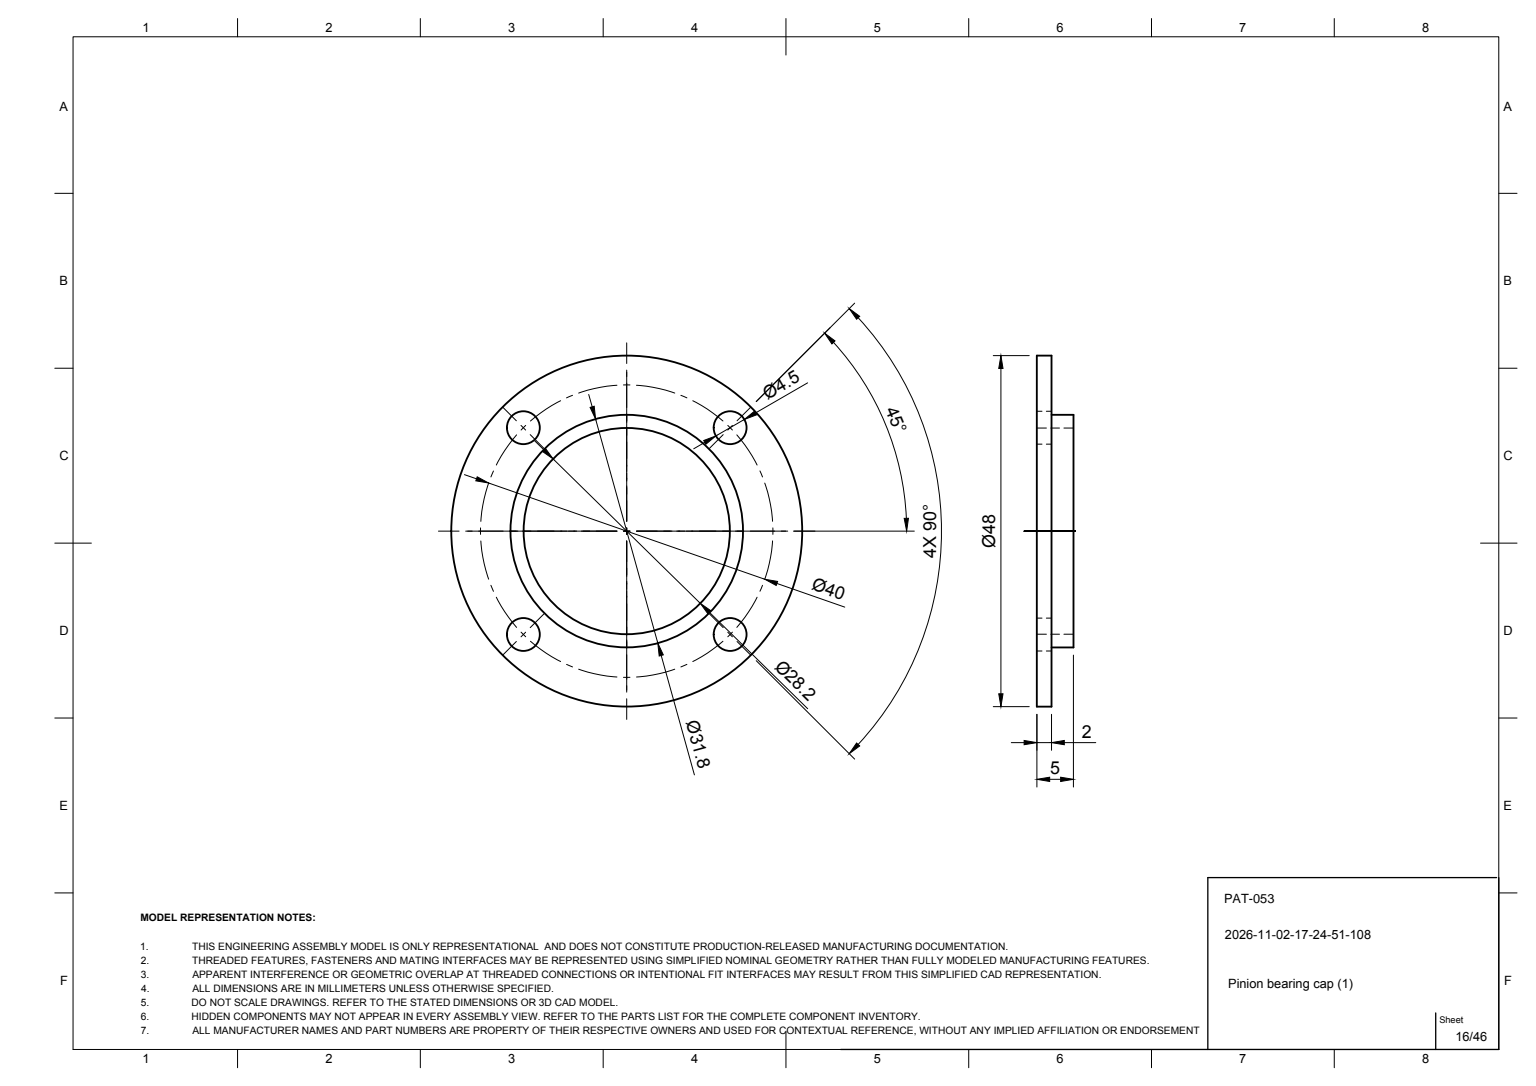
ISO-10303-21;
HEADER;
/* Generated by software containing ST-Developer
 * from STEP Tools, Inc. (www.steptools.com) 
 */

FILE_DESCRIPTION(
/* description */ ('Hand-operated arbor press'),
/* implementation_level */ '2;1');

FILE_NAME(
/* name */ 'Pinion bearing cap (1).step',
/* time_stamp */ '2026-10-28T03:25:25-07:00',
/* author */ (''),
/* organization */ (''),
/* preprocessor_version */ 'ST-DEVELOPER v20.2',
/* originating_system */ 'Autodesk Translation Framework v15.17.0.0',
/* authorisation */ '');

FILE_SCHEMA (('AUTOMOTIVE_DESIGN { 1 0 10303 214 3 1 1 }'));
ENDSEC;

DATA;
#10=MECHANICAL_DESIGN_GEOMETRIC_PRESENTATION_REPRESENTATION('',(#597),#32751);
#513=SHAPE_REPRESENTATION_RELATIONSHIP('SRR','None',#32942,#555);
#555=ADVANCED_BREP_SHAPE_REPRESENTATION('',(#646),#32716);
#597=STYLED_ITEM('',(#33242),#646);
#646=MANIFOLD_SOLID_BREP('Body1',#12494);
#754=FACE_BOUND('',#2209,.T.);
#755=FACE_BOUND('',#2212,.T.);
#756=FACE_BOUND('',#2213,.T.);
#757=FACE_BOUND('',#2214,.T.);
#758=FACE_BOUND('',#2215,.T.);
#759=FACE_BOUND('',#2216,.T.);
#760=FACE_BOUND('',#2218,.T.);
#761=FACE_BOUND('',#2219,.T.);
#762=FACE_BOUND('',#2220,.T.);
#763=FACE_BOUND('',#2221,.T.);
#764=FACE_BOUND('',#2222,.T.);
#947=PLANE('',#13297);
#948=PLANE('',#13301);
#949=PLANE('',#13302);
#1447=FACE_OUTER_BOUND('',#2202,.T.);
#1448=FACE_OUTER_BOUND('',#2203,.T.);
#1449=FACE_OUTER_BOUND('',#2204,.T.);
#1450=FACE_OUTER_BOUND('',#2205,.T.);
#1451=FACE_OUTER_BOUND('',#2206,.T.);
#1452=FACE_OUTER_BOUND('',#2207,.T.);
#1453=FACE_OUTER_BOUND('',#2208,.T.);
#1454=FACE_OUTER_BOUND('',#2210,.T.);
#1455=FACE_OUTER_BOUND('',#2211,.T.);
#1456=FACE_OUTER_BOUND('',#2217,.T.);
#2202=EDGE_LOOP('',(#9056,#9057,#9058,#9059));
#2203=EDGE_LOOP('',(#9060,#9061,#9062,#9063));
#2204=EDGE_LOOP('',(#9064,#9065,#9066,#9067));
#2205=EDGE_LOOP('',(#9068,#9069,#9070,#9071));
#2206=EDGE_LOOP('',(#9072,#9073,#9074,#9075));
#2207=EDGE_LOOP('',(#9076,#9077,#9078,#9079));
#2208=EDGE_LOOP('',(#9080));
#2209=EDGE_LOOP('',(#9081));
#2210=EDGE_LOOP('',(#9082,#9083,#9084,#9085));
#2211=EDGE_LOOP('',(#9086));
#2212=EDGE_LOOP('',(#9087));
#2213=EDGE_LOOP('',(#9088));
#2214=EDGE_LOOP('',(#9089));
#2215=EDGE_LOOP('',(#9090));
#2216=EDGE_LOOP('',(#9091));
#2217=EDGE_LOOP('',(#9092));
#2218=EDGE_LOOP('',(#9093));
#2219=EDGE_LOOP('',(#9094));
#2220=EDGE_LOOP('',(#9095));
#2221=EDGE_LOOP('',(#9096));
#2222=EDGE_LOOP('',(#9097));
#3078=LINE('',#18420,#4249);
#3079=LINE('',#18426,#4250);
#3080=LINE('',#18432,#4251);
#3081=LINE('',#18438,#4252);
#3082=LINE('',#18444,#4253);
#3083=LINE('',#18450,#4254);
#3084=LINE('',#18457,#4255);
#4249=VECTOR('',#14973,1.41);
#4250=VECTOR('',#14980,0.225);
#4251=VECTOR('',#14987,0.225);
#4252=VECTOR('',#14994,0.225);
#4253=VECTOR('',#15001,0.225);
#4254=VECTOR('',#15008,1.59);
#4255=VECTOR('',#15017,2.4);
#5278=CIRCLE('',#13280,1.41);
#5279=CIRCLE('',#13281,1.41);
#5280=CIRCLE('',#13283,0.225);
#5281=CIRCLE('',#13284,0.225);
#5282=CIRCLE('',#13286,0.225);
#5283=CIRCLE('',#13287,0.225);
#5284=CIRCLE('',#13289,0.225);
#5285=CIRCLE('',#13290,0.225);
#5286=CIRCLE('',#13292,0.225);
#5287=CIRCLE('',#13293,0.225);
#5288=CIRCLE('',#13295,1.59);
#5289=CIRCLE('',#13296,1.59);
#5290=CIRCLE('',#13299,2.4);
#5291=CIRCLE('',#13300,2.4);
#5800=VERTEX_POINT('',#18417);
#5801=VERTEX_POINT('',#18419);
#5802=VERTEX_POINT('',#18423);
#5803=VERTEX_POINT('',#18425);
#5804=VERTEX_POINT('',#18429);
#5805=VERTEX_POINT('',#18431);
#5806=VERTEX_POINT('',#18435);
#5807=VERTEX_POINT('',#18437);
#5808=VERTEX_POINT('',#18441);
#5809=VERTEX_POINT('',#18443);
#5810=VERTEX_POINT('',#18447);
#5811=VERTEX_POINT('',#18449);
#5812=VERTEX_POINT('',#18454);
#5813=VERTEX_POINT('',#18456);
#7031=EDGE_CURVE('',#5800,#5800,#5278,.T.);
#7032=EDGE_CURVE('',#5800,#5801,#3078,.T.);
#7033=EDGE_CURVE('',#5801,#5801,#5279,.T.);
#7034=EDGE_CURVE('',#5802,#5802,#5280,.T.);
#7035=EDGE_CURVE('',#5802,#5803,#3079,.T.);
#7036=EDGE_CURVE('',#5803,#5803,#5281,.T.);
#7037=EDGE_CURVE('',#5804,#5804,#5282,.T.);
#7038=EDGE_CURVE('',#5804,#5805,#3080,.T.);
#7039=EDGE_CURVE('',#5805,#5805,#5283,.T.);
#7040=EDGE_CURVE('',#5806,#5806,#5284,.T.);
#7041=EDGE_CURVE('',#5806,#5807,#3081,.T.);
#7042=EDGE_CURVE('',#5807,#5807,#5285,.T.);
#7043=EDGE_CURVE('',#5808,#5808,#5286,.T.);
#7044=EDGE_CURVE('',#5808,#5809,#3082,.T.);
#7045=EDGE_CURVE('',#5809,#5809,#5287,.T.);
#7046=EDGE_CURVE('',#5810,#5810,#5288,.T.);
#7047=EDGE_CURVE('',#5810,#5811,#3083,.T.);
#7048=EDGE_CURVE('',#5811,#5811,#5289,.T.);
#7049=EDGE_CURVE('',#5812,#5812,#5290,.T.);
#7050=EDGE_CURVE('',#5812,#5813,#3084,.T.);
#7051=EDGE_CURVE('',#5813,#5813,#5291,.T.);
#9056=ORIENTED_EDGE('',*,*,#7031,.F.);
#9057=ORIENTED_EDGE('',*,*,#7032,.T.);
#9058=ORIENTED_EDGE('',*,*,#7033,.F.);
#9059=ORIENTED_EDGE('',*,*,#7032,.F.);
#9060=ORIENTED_EDGE('',*,*,#7034,.F.);
#9061=ORIENTED_EDGE('',*,*,#7035,.T.);
#9062=ORIENTED_EDGE('',*,*,#7036,.F.);
#9063=ORIENTED_EDGE('',*,*,#7035,.F.);
#9064=ORIENTED_EDGE('',*,*,#7037,.F.);
#9065=ORIENTED_EDGE('',*,*,#7038,.T.);
#9066=ORIENTED_EDGE('',*,*,#7039,.F.);
#9067=ORIENTED_EDGE('',*,*,#7038,.F.);
#9068=ORIENTED_EDGE('',*,*,#7040,.F.);
#9069=ORIENTED_EDGE('',*,*,#7041,.T.);
#9070=ORIENTED_EDGE('',*,*,#7042,.F.);
#9071=ORIENTED_EDGE('',*,*,#7041,.F.);
#9072=ORIENTED_EDGE('',*,*,#7043,.F.);
#9073=ORIENTED_EDGE('',*,*,#7044,.T.);
#9074=ORIENTED_EDGE('',*,*,#7045,.F.);
#9075=ORIENTED_EDGE('',*,*,#7044,.F.);
#9076=ORIENTED_EDGE('',*,*,#7046,.F.);
#9077=ORIENTED_EDGE('',*,*,#7047,.T.);
#9078=ORIENTED_EDGE('',*,*,#7048,.T.);
#9079=ORIENTED_EDGE('',*,*,#7047,.F.);
#9080=ORIENTED_EDGE('',*,*,#7048,.F.);
#9081=ORIENTED_EDGE('',*,*,#7031,.T.);
#9082=ORIENTED_EDGE('',*,*,#7049,.F.);
#9083=ORIENTED_EDGE('',*,*,#7050,.T.);
#9084=ORIENTED_EDGE('',*,*,#7051,.T.);
#9085=ORIENTED_EDGE('',*,*,#7050,.F.);
#9086=ORIENTED_EDGE('',*,*,#7049,.T.);
#9087=ORIENTED_EDGE('',*,*,#7033,.T.);
#9088=ORIENTED_EDGE('',*,*,#7045,.T.);
#9089=ORIENTED_EDGE('',*,*,#7042,.T.);
#9090=ORIENTED_EDGE('',*,*,#7039,.T.);
#9091=ORIENTED_EDGE('',*,*,#7036,.T.);
#9092=ORIENTED_EDGE('',*,*,#7051,.F.);
#9093=ORIENTED_EDGE('',*,*,#7046,.T.);
#9094=ORIENTED_EDGE('',*,*,#7043,.T.);
#9095=ORIENTED_EDGE('',*,*,#7040,.T.);
#9096=ORIENTED_EDGE('',*,*,#7037,.T.);
#9097=ORIENTED_EDGE('',*,*,#7034,.T.);
#11698=CYLINDRICAL_SURFACE('',#13279,1.41);
#11699=CYLINDRICAL_SURFACE('',#13282,0.225);
#11700=CYLINDRICAL_SURFACE('',#13285,0.225);
#11701=CYLINDRICAL_SURFACE('',#13288,0.225);
#11702=CYLINDRICAL_SURFACE('',#13291,0.225);
#11703=CYLINDRICAL_SURFACE('',#13294,1.59);
#11704=CYLINDRICAL_SURFACE('',#13298,2.4);
#11956=ADVANCED_FACE('',(#1447),#11698,.F.);
#11957=ADVANCED_FACE('',(#1448),#11699,.F.);
#11958=ADVANCED_FACE('',(#1449),#11700,.F.);
#11959=ADVANCED_FACE('',(#1450),#11701,.F.);
#11960=ADVANCED_FACE('',(#1451),#11702,.F.);
#11961=ADVANCED_FACE('',(#1452),#11703,.T.);
#11962=ADVANCED_FACE('',(#1453,#754),#947,.F.);
#11963=ADVANCED_FACE('',(#1454),#11704,.T.);
#11964=ADVANCED_FACE('',(#1455,#755,#756,#757,#758,#759),#948,.T.);
#11965=ADVANCED_FACE('',(#1456,#760,#761,#762,#763,#764),#949,.F.);
#12494=CLOSED_SHELL('',(#11956,#11957,#11958,#11959,#11960,#11961,#11962,
#11963,#11964,#11965));
#13278=AXIS2_PLACEMENT_3D('',#18415,#14967,#14968);
#13279=AXIS2_PLACEMENT_3D('',#18416,#14969,#14970);
#13280=AXIS2_PLACEMENT_3D('',#18418,#14971,#14972);
#13281=AXIS2_PLACEMENT_3D('',#18421,#14974,#14975);
#13282=AXIS2_PLACEMENT_3D('',#18422,#14976,#14977);
#13283=AXIS2_PLACEMENT_3D('',#18424,#14978,#14979);
#13284=AXIS2_PLACEMENT_3D('',#18427,#14981,#14982);
#13285=AXIS2_PLACEMENT_3D('',#18428,#14983,#14984);
#13286=AXIS2_PLACEMENT_3D('',#18430,#14985,#14986);
#13287=AXIS2_PLACEMENT_3D('',#18433,#14988,#14989);
#13288=AXIS2_PLACEMENT_3D('',#18434,#14990,#14991);
#13289=AXIS2_PLACEMENT_3D('',#18436,#14992,#14993);
#13290=AXIS2_PLACEMENT_3D('',#18439,#14995,#14996);
#13291=AXIS2_PLACEMENT_3D('',#18440,#14997,#14998);
#13292=AXIS2_PLACEMENT_3D('',#18442,#14999,#15000);
#13293=AXIS2_PLACEMENT_3D('',#18445,#15002,#15003);
#13294=AXIS2_PLACEMENT_3D('',#18446,#15004,#15005);
#13295=AXIS2_PLACEMENT_3D('',#18448,#15006,#15007);
#13296=AXIS2_PLACEMENT_3D('',#18451,#15009,#15010);
#13297=AXIS2_PLACEMENT_3D('',#18452,#15011,#15012);
#13298=AXIS2_PLACEMENT_3D('',#18453,#15013,#15014);
#13299=AXIS2_PLACEMENT_3D('',#18455,#15015,#15016);
#13300=AXIS2_PLACEMENT_3D('',#18458,#15018,#15019);
#13301=AXIS2_PLACEMENT_3D('',#18459,#15020,#15021);
#13302=AXIS2_PLACEMENT_3D('',#18460,#15022,#15023);
#14967=DIRECTION('axis',(0.,0.,1.));
#14968=DIRECTION('refdir',(1.,0.,0.));
#14969=DIRECTION('center_axis',(0.,1.,0.));
#14970=DIRECTION('ref_axis',(1.,0.,0.));
#14971=DIRECTION('center_axis',(0.,1.,0.));
#14972=DIRECTION('ref_axis',(1.,0.,0.));
#14973=DIRECTION('',(0.,1.,0.));
#14974=DIRECTION('center_axis',(0.,-1.,0.));
#14975=DIRECTION('ref_axis',(1.,0.,0.));
#14976=DIRECTION('center_axis',(0.,1.,0.));
#14977=DIRECTION('ref_axis',(1.,0.,0.));
#14978=DIRECTION('center_axis',(0.,1.,0.));
#14979=DIRECTION('ref_axis',(1.,0.,0.));
#14980=DIRECTION('',(0.,1.,0.));
#14981=DIRECTION('center_axis',(0.,-1.,0.));
#14982=DIRECTION('ref_axis',(1.,0.,0.));
#14983=DIRECTION('center_axis',(0.,1.,0.));
#14984=DIRECTION('ref_axis',(1.,0.,0.));
#14985=DIRECTION('center_axis',(0.,1.,0.));
#14986=DIRECTION('ref_axis',(1.,0.,0.));
#14987=DIRECTION('',(0.,1.,0.));
#14988=DIRECTION('center_axis',(0.,-1.,0.));
#14989=DIRECTION('ref_axis',(1.,0.,0.));
#14990=DIRECTION('center_axis',(0.,1.,0.));
#14991=DIRECTION('ref_axis',(1.,0.,0.));
#14992=DIRECTION('center_axis',(0.,1.,0.));
#14993=DIRECTION('ref_axis',(1.,0.,0.));
#14994=DIRECTION('',(0.,1.,0.));
#14995=DIRECTION('center_axis',(0.,-1.,0.));
#14996=DIRECTION('ref_axis',(1.,0.,0.));
#14997=DIRECTION('center_axis',(0.,1.,0.));
#14998=DIRECTION('ref_axis',(1.,0.,0.));
#14999=DIRECTION('center_axis',(0.,1.,0.));
#15000=DIRECTION('ref_axis',(1.,0.,0.));
#15001=DIRECTION('',(0.,1.,0.));
#15002=DIRECTION('center_axis',(0.,-1.,0.));
#15003=DIRECTION('ref_axis',(1.,0.,0.));
#15004=DIRECTION('center_axis',(0.,1.,0.));
#15005=DIRECTION('ref_axis',(1.,0.,0.));
#15006=DIRECTION('center_axis',(0.,1.,0.));
#15007=DIRECTION('ref_axis',(1.,0.,0.));
#15008=DIRECTION('',(0.,-1.,0.));
#15009=DIRECTION('center_axis',(0.,1.,0.));
#15010=DIRECTION('ref_axis',(1.,0.,0.));
#15011=DIRECTION('center_axis',(0.,1.,0.));
#15012=DIRECTION('ref_axis',(1.,0.,0.));
#15013=DIRECTION('center_axis',(0.,1.,0.));
#15014=DIRECTION('ref_axis',(1.,0.,0.));
#15015=DIRECTION('center_axis',(0.,1.,0.));
#15016=DIRECTION('ref_axis',(1.,0.,0.));
#15017=DIRECTION('',(0.,-1.,0.));
#15018=DIRECTION('center_axis',(0.,1.,0.));
#15019=DIRECTION('ref_axis',(1.,0.,0.));
#15020=DIRECTION('center_axis',(0.,1.,0.));
#15021=DIRECTION('ref_axis',(1.,0.,0.));
#15022=DIRECTION('center_axis',(0.,1.,0.));
#15023=DIRECTION('ref_axis',(1.,0.,0.));
#18415=CARTESIAN_POINT('',(0.,0.,0.));
#18416=CARTESIAN_POINT('Origin',(-3.25,-4.1,20.));
#18417=CARTESIAN_POINT('',(-4.66,-2.5,20.));
#18418=CARTESIAN_POINT('Origin',(-3.25,-2.5,20.));
#18419=CARTESIAN_POINT('',(-4.66,-2.,20.));
#18420=CARTESIAN_POINT('',(-4.66,-4.1,20.));
#18421=CARTESIAN_POINT('Origin',(-3.25,-2.,20.));
#18422=CARTESIAN_POINT('Origin',(-4.66421356237309,-2.3,18.5857864376269));
#18423=CARTESIAN_POINT('',(-4.88921356237309,-2.2,18.5857864376269));
#18424=CARTESIAN_POINT('Origin',(-4.66421356237309,-2.2,18.5857864376269));
#18425=CARTESIAN_POINT('',(-4.88921356237309,-2.,18.5857864376269));
#18426=CARTESIAN_POINT('',(-4.88921356237309,-2.3,18.5857864376269));
#18427=CARTESIAN_POINT('Origin',(-4.66421356237309,-2.,18.5857864376269));
#18428=CARTESIAN_POINT('Origin',(-4.66421356237309,-2.3,21.4142135623731));
#18429=CARTESIAN_POINT('',(-4.88921356237309,-2.2,21.4142135623731));
#18430=CARTESIAN_POINT('Origin',(-4.66421356237309,-2.2,21.4142135623731));
#18431=CARTESIAN_POINT('',(-4.88921356237309,-2.,21.4142135623731));
#18432=CARTESIAN_POINT('',(-4.88921356237309,-2.3,21.4142135623731));
#18433=CARTESIAN_POINT('Origin',(-4.66421356237309,-2.,21.4142135623731));
#18434=CARTESIAN_POINT('Origin',(-1.8357864376269,-2.3,21.4142135623731));
#18435=CARTESIAN_POINT('',(-2.0607864376269,-2.2,21.4142135623731));
#18436=CARTESIAN_POINT('Origin',(-1.8357864376269,-2.2,21.4142135623731));
#18437=CARTESIAN_POINT('',(-2.0607864376269,-2.,21.4142135623731));
#18438=CARTESIAN_POINT('',(-2.0607864376269,-2.3,21.4142135623731));
#18439=CARTESIAN_POINT('Origin',(-1.8357864376269,-2.,21.4142135623731));
#18440=CARTESIAN_POINT('Origin',(-1.83578643762691,-2.3,18.5857864376269));
#18441=CARTESIAN_POINT('',(-2.06078643762691,-2.2,18.5857864376269));
#18442=CARTESIAN_POINT('Origin',(-1.83578643762691,-2.2,18.5857864376269));
#18443=CARTESIAN_POINT('',(-2.06078643762691,-2.,18.5857864376269));
#18444=CARTESIAN_POINT('',(-2.06078643762691,-2.3,18.5857864376269));
#18445=CARTESIAN_POINT('Origin',(-1.83578643762691,-2.,18.5857864376269));
#18446=CARTESIAN_POINT('Origin',(-3.25,-2.5,20.));
#18447=CARTESIAN_POINT('',(-4.84,-2.2,20.));
#18448=CARTESIAN_POINT('Origin',(-3.25,-2.2,20.));
#18449=CARTESIAN_POINT('',(-4.84,-2.5,20.));
#18450=CARTESIAN_POINT('',(-4.84,-2.5,20.));
#18451=CARTESIAN_POINT('Origin',(-3.25,-2.5,20.));
#18452=CARTESIAN_POINT('Origin',(-3.25,-2.5,20.));
#18453=CARTESIAN_POINT('Origin',(-3.25,-2.2,20.));
#18454=CARTESIAN_POINT('',(-5.65,-2.,20.));
#18455=CARTESIAN_POINT('Origin',(-3.25,-2.,20.));
#18456=CARTESIAN_POINT('',(-5.65,-2.2,20.));
#18457=CARTESIAN_POINT('',(-5.65,-2.2,20.));
#18458=CARTESIAN_POINT('Origin',(-3.25,-2.2,20.));
#18459=CARTESIAN_POINT('Origin',(-3.25,-2.,20.));
#18460=CARTESIAN_POINT('Origin',(-3.25,-2.2,20.));
#32667=UNCERTAINTY_MEASURE_WITH_UNIT(LENGTH_MEASURE(0.001),#32752,
'DISTANCE_ACCURACY_VALUE',
'Maximum model space distance between geometric entities at asserted c
onnectivities');
#32702=UNCERTAINTY_MEASURE_WITH_UNIT(LENGTH_MEASURE(0.001),#32752,
'DISTANCE_ACCURACY_VALUE',
'Maximum model space distance between geometric entities at asserted c
onnectivities');
#32716=(
GEOMETRIC_REPRESENTATION_CONTEXT(3)
GLOBAL_UNCERTAINTY_ASSIGNED_CONTEXT((#32667))
GLOBAL_UNIT_ASSIGNED_CONTEXT((#32752,#32754,#32755))
REPRESENTATION_CONTEXT('','3D')
);
#32751=(
GEOMETRIC_REPRESENTATION_CONTEXT(3)
GLOBAL_UNCERTAINTY_ASSIGNED_CONTEXT((#32702))
GLOBAL_UNIT_ASSIGNED_CONTEXT((#32752,#32754,#32755))
REPRESENTATION_CONTEXT('','3D')
);
#32752=(
LENGTH_UNIT()
NAMED_UNIT(*)
SI_UNIT(.CENTI.,.METRE.)
);
#32754=(
NAMED_UNIT(*)
PLANE_ANGLE_UNIT()
SI_UNIT($,.RADIAN.)
);
#32755=(
NAMED_UNIT(*)
SI_UNIT($,.STERADIAN.)
SOLID_ANGLE_UNIT()
);
#32769=SHAPE_DEFINITION_REPRESENTATION(#32817,#32942);
#32817=PRODUCT_DEFINITION_SHAPE('',$,#32991);
#32942=SHAPE_REPRESENTATION('',(#13278),#32716);
#32977=PRODUCT_DEFINITION_CONTEXT('part definition',#33123,'design');
#32991=PRODUCT_DEFINITION('Pinion bearing cap (1)',
'Pinion bearing cap (1)',#33039,#32977);
#33039=PRODUCT_DEFINITION_FORMATION('',$,#33138);
#33123=APPLICATION_CONTEXT(
'Core Data for Automotive Mechanical Design Process');
#33124=PRODUCT_CONTEXT('part definition',#33123,'mechanical');
#33138=PRODUCT('Pinion bearing cap (1)','Pinion bearing cap (1)',
'Pinion bearing cap (1)',(#33124));
#33236=COLOUR_RGB('Grey',0.48,0.52,0.57);
#33237=FILL_AREA_STYLE_COLOUR('',#33236);
#33238=FILL_AREA_STYLE('',(#33237));
#33239=SURFACE_STYLE_FILL_AREA(#33238);
#33240=SURFACE_SIDE_STYLE('',(#33239));
#33241=SURFACE_STYLE_USAGE(.BOTH.,#33240);
#33242=PRESENTATION_STYLE_ASSIGNMENT((#33241));
ENDSEC;
END-ISO-10303-21;
